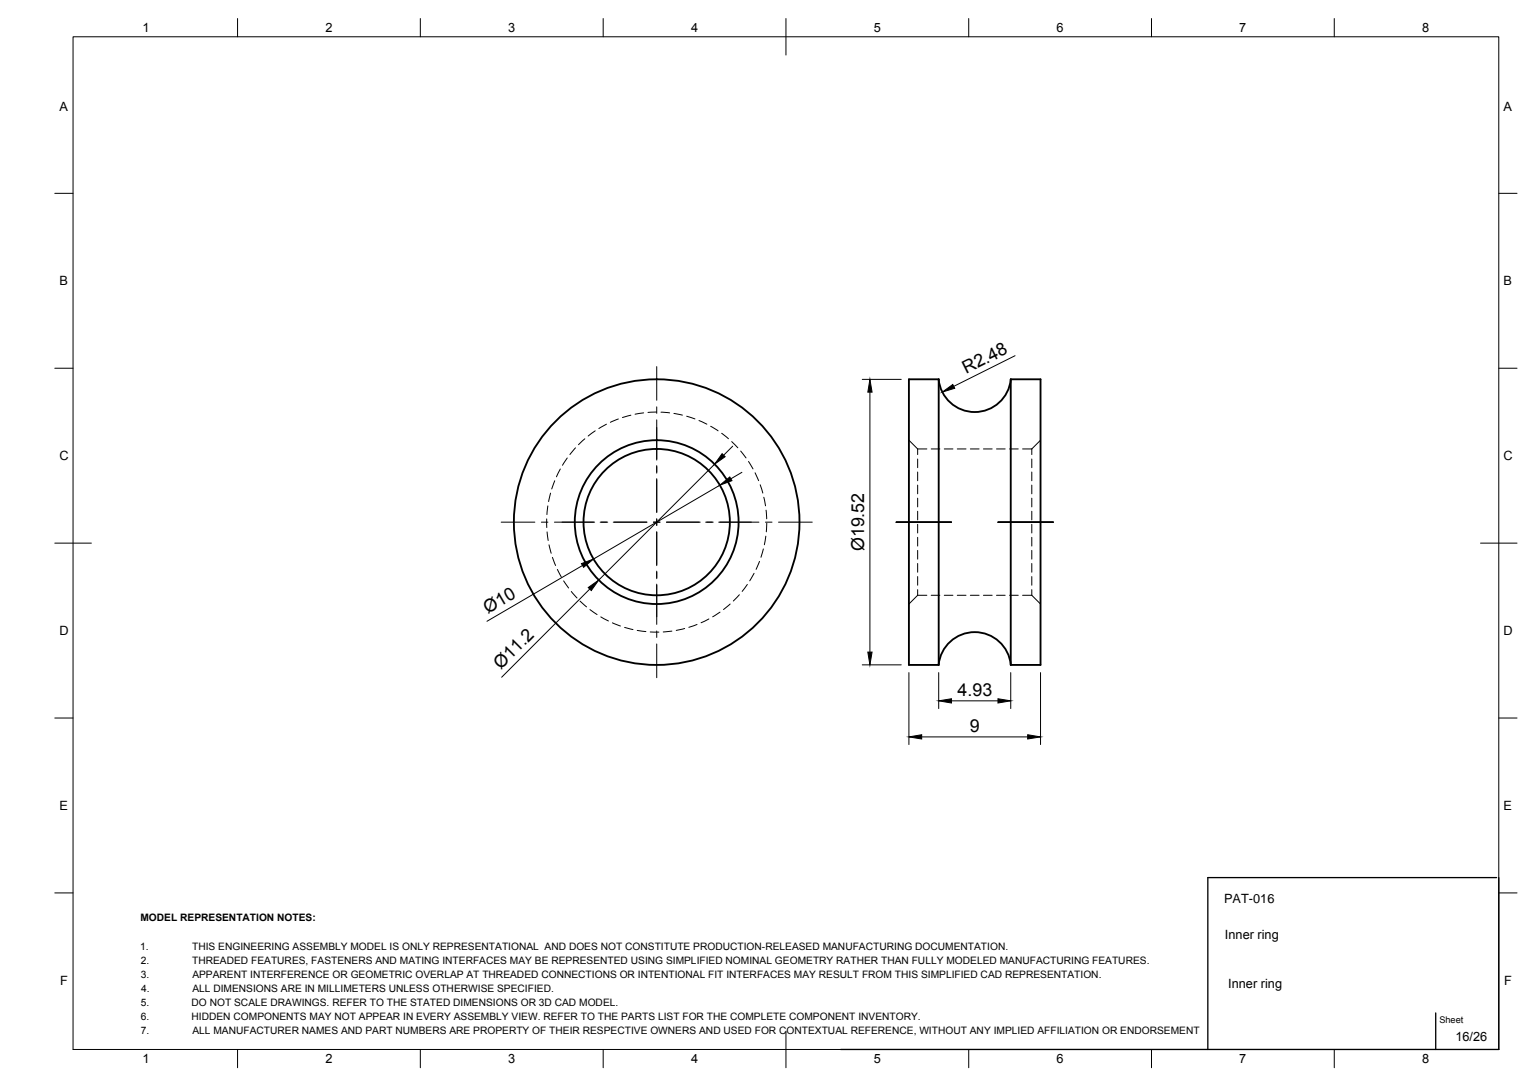
ISO-10303-21;
HEADER;
/* Generated by software containing ST-Developer
 * from STEP Tools, Inc. (www.steptools.com) 
 */

FILE_DESCRIPTION(
/* description */ ('Bracket-mounted idler roller'),
/* implementation_level */ '2;1');

FILE_NAME(
/* name */ 'Inner ring.step',
/* time_stamp */ '2026-10-28T03:26:42-07:00',
/* author */ (''),
/* organization */ (''),
/* preprocessor_version */ 'ST-DEVELOPER v20.2',
/* originating_system */ 'Autodesk Translation Framework v15.17.0.0',
/* authorisation */ '');

FILE_SCHEMA (('AUTOMOTIVE_DESIGN { 1 0 10303 214 3 1 1 }'));
ENDSEC;

DATA;
#10=MECHANICAL_DESIGN_GEOMETRIC_PRESENTATION_REPRESENTATION('',(#291),#6241);
#221=TOROIDAL_SURFACE('',#3608,1.,0.247676);
#226=CONICAL_SURFACE('',#3619,0.53,0.785398163397448);
#227=CONICAL_SURFACE('',#3626,0.53,0.785398163397448);
#249=SHAPE_REPRESENTATION_RELATIONSHIP('SRR','None',#6354,#270);
#270=ADVANCED_BREP_SHAPE_REPRESENTATION('',(#319),#6230);
#291=STYLED_ITEM('',(#6538),#319);
#319=MANIFOLD_SOLID_BREP('Body1',#3194);
#373=FACE_BOUND('',#840,.T.);
#374=FACE_BOUND('',#843,.T.);
#478=PLANE('',#3621);
#479=PLANE('',#3624);
#607=FACE_OUTER_BOUND('',#835,.T.);
#608=FACE_OUTER_BOUND('',#836,.T.);
#609=FACE_OUTER_BOUND('',#837,.T.);
#610=FACE_OUTER_BOUND('',#838,.T.);
#611=FACE_OUTER_BOUND('',#839,.T.);
#612=FACE_OUTER_BOUND('',#841,.T.);
#613=FACE_OUTER_BOUND('',#842,.T.);
#614=FACE_OUTER_BOUND('',#844,.T.);
#835=EDGE_LOOP('',(#2520,#2521,#2522,#2523,#2524,#2525));
#836=EDGE_LOOP('',(#2526,#2527,#2528,#2529,#2530));
#837=EDGE_LOOP('',(#2531,#2532,#2533,#2534));
#838=EDGE_LOOP('',(#2535,#2536,#2537,#2538));
#839=EDGE_LOOP('',(#2539));
#840=EDGE_LOOP('',(#2540));
#841=EDGE_LOOP('',(#2541,#2542,#2543,#2544,#2545));
#842=EDGE_LOOP('',(#2546));
#843=EDGE_LOOP('',(#2547));
#844=EDGE_LOOP('',(#2548,#2549,#2550,#2551));
#1099=LINE('',#5362,#1281);
#1100=LINE('',#5368,#1282);
#1101=LINE('',#5372,#1283);
#1102=LINE('',#5378,#1284);
#1103=LINE('',#5383,#1285);
#1281=VECTOR('',#4346,0.976185);
#1282=VECTOR('',#4353,0.5);
#1283=VECTOR('',#4358,0.53);
#1284=VECTOR('',#4367,0.976185);
#1285=VECTOR('',#4374,0.53);
#1400=CIRCLE('',#3609,0.976185);
#1401=CIRCLE('',#3610,0.976185);
#1402=CIRCLE('',#3611,0.247676);
#1403=CIRCLE('',#3612,0.976185);
#1404=CIRCLE('',#3613,0.976185);
#1405=CIRCLE('',#3615,0.976185);
#1406=CIRCLE('',#3617,0.5);
#1407=CIRCLE('',#3618,0.5);
#1408=CIRCLE('',#3620,0.56);
#1409=CIRCLE('',#3623,0.976185);
#1410=CIRCLE('',#3625,0.56);
#1641=VERTEX_POINT('',#5351);
#1642=VERTEX_POINT('',#5352);
#1643=VERTEX_POINT('',#5355);
#1644=VERTEX_POINT('',#5357);
#1645=VERTEX_POINT('',#5361);
#1646=VERTEX_POINT('',#5365);
#1647=VERTEX_POINT('',#5367);
#1648=VERTEX_POINT('',#5371);
#1649=VERTEX_POINT('',#5376);
#1650=VERTEX_POINT('',#5380);
#1962=EDGE_CURVE('',#1641,#1642,#1400,.T.);
#1963=EDGE_CURVE('',#1642,#1641,#1401,.T.);
#1964=EDGE_CURVE('',#1642,#1643,#1402,.T.);
#1965=EDGE_CURVE('',#1644,#1643,#1403,.T.);
#1966=EDGE_CURVE('',#1643,#1644,#1404,.T.);
#1967=EDGE_CURVE('',#1644,#1645,#1099,.T.);
#1968=EDGE_CURVE('',#1645,#1645,#1405,.T.);
#1969=EDGE_CURVE('',#1646,#1646,#1406,.T.);
#1970=EDGE_CURVE('',#1646,#1647,#1100,.T.);
#1971=EDGE_CURVE('',#1647,#1647,#1407,.T.);
#1972=EDGE_CURVE('',#1647,#1648,#1101,.T.);
#1973=EDGE_CURVE('',#1648,#1648,#1408,.T.);
#1974=EDGE_CURVE('',#1649,#1649,#1409,.T.);
#1975=EDGE_CURVE('',#1649,#1641,#1102,.T.);
#1976=EDGE_CURVE('',#1650,#1650,#1410,.T.);
#1977=EDGE_CURVE('',#1650,#1646,#1103,.T.);
#2520=ORIENTED_EDGE('',*,*,#1962,.F.);
#2521=ORIENTED_EDGE('',*,*,#1963,.F.);
#2522=ORIENTED_EDGE('',*,*,#1964,.T.);
#2523=ORIENTED_EDGE('',*,*,#1965,.F.);
#2524=ORIENTED_EDGE('',*,*,#1966,.F.);
#2525=ORIENTED_EDGE('',*,*,#1964,.F.);
#2526=ORIENTED_EDGE('',*,*,#1965,.T.);
#2527=ORIENTED_EDGE('',*,*,#1966,.T.);
#2528=ORIENTED_EDGE('',*,*,#1967,.T.);
#2529=ORIENTED_EDGE('',*,*,#1968,.T.);
#2530=ORIENTED_EDGE('',*,*,#1967,.F.);
#2531=ORIENTED_EDGE('',*,*,#1969,.T.);
#2532=ORIENTED_EDGE('',*,*,#1970,.T.);
#2533=ORIENTED_EDGE('',*,*,#1971,.F.);
#2534=ORIENTED_EDGE('',*,*,#1970,.F.);
#2535=ORIENTED_EDGE('',*,*,#1971,.T.);
#2536=ORIENTED_EDGE('',*,*,#1972,.T.);
#2537=ORIENTED_EDGE('',*,*,#1973,.F.);
#2538=ORIENTED_EDGE('',*,*,#1972,.F.);
#2539=ORIENTED_EDGE('',*,*,#1968,.F.);
#2540=ORIENTED_EDGE('',*,*,#1973,.T.);
#2541=ORIENTED_EDGE('',*,*,#1974,.F.);
#2542=ORIENTED_EDGE('',*,*,#1975,.T.);
#2543=ORIENTED_EDGE('',*,*,#1962,.T.);
#2544=ORIENTED_EDGE('',*,*,#1963,.T.);
#2545=ORIENTED_EDGE('',*,*,#1975,.F.);
#2546=ORIENTED_EDGE('',*,*,#1974,.T.);
#2547=ORIENTED_EDGE('',*,*,#1976,.F.);
#2548=ORIENTED_EDGE('',*,*,#1976,.T.);
#2549=ORIENTED_EDGE('',*,*,#1977,.T.);
#2550=ORIENTED_EDGE('',*,*,#1969,.F.);
#2551=ORIENTED_EDGE('',*,*,#1977,.F.);
#2955=CYLINDRICAL_SURFACE('',#3614,0.976185);
#2956=CYLINDRICAL_SURFACE('',#3616,0.5);
#2957=CYLINDRICAL_SURFACE('',#3622,0.976185);
#3082=ADVANCED_FACE('',(#607),#221,.F.);
#3083=ADVANCED_FACE('',(#608),#2955,.T.);
#3084=ADVANCED_FACE('',(#609),#2956,.F.);
#3085=ADVANCED_FACE('',(#610),#226,.F.);
#3086=ADVANCED_FACE('',(#611,#373),#478,.T.);
#3087=ADVANCED_FACE('',(#612),#2957,.T.);
#3088=ADVANCED_FACE('',(#613,#374),#479,.T.);
#3089=ADVANCED_FACE('',(#614),#227,.F.);
#3194=CLOSED_SHELL('',(#3082,#3083,#3084,#3085,#3086,#3087,#3088,#3089));
#3607=AXIS2_PLACEMENT_3D('',#5349,#4330,#4331);
#3608=AXIS2_PLACEMENT_3D('',#5350,#4332,#4333);
#3609=AXIS2_PLACEMENT_3D('',#5353,#4334,#4335);
#3610=AXIS2_PLACEMENT_3D('',#5354,#4336,#4337);
#3611=AXIS2_PLACEMENT_3D('',#5356,#4338,#4339);
#3612=AXIS2_PLACEMENT_3D('',#5358,#4340,#4341);
#3613=AXIS2_PLACEMENT_3D('',#5359,#4342,#4343);
#3614=AXIS2_PLACEMENT_3D('',#5360,#4344,#4345);
#3615=AXIS2_PLACEMENT_3D('',#5363,#4347,#4348);
#3616=AXIS2_PLACEMENT_3D('',#5364,#4349,#4350);
#3617=AXIS2_PLACEMENT_3D('',#5366,#4351,#4352);
#3618=AXIS2_PLACEMENT_3D('',#5369,#4354,#4355);
#3619=AXIS2_PLACEMENT_3D('',#5370,#4356,#4357);
#3620=AXIS2_PLACEMENT_3D('',#5373,#4359,#4360);
#3621=AXIS2_PLACEMENT_3D('',#5374,#4361,#4362);
#3622=AXIS2_PLACEMENT_3D('',#5375,#4363,#4364);
#3623=AXIS2_PLACEMENT_3D('',#5377,#4365,#4366);
#3624=AXIS2_PLACEMENT_3D('',#5379,#4368,#4369);
#3625=AXIS2_PLACEMENT_3D('',#5381,#4370,#4371);
#3626=AXIS2_PLACEMENT_3D('',#5382,#4372,#4373);
#4330=DIRECTION('axis',(0.,0.,1.));
#4331=DIRECTION('refdir',(1.,0.,0.));
#4332=DIRECTION('center_axis',(0.,-1.,0.));
#4333=DIRECTION('ref_axis',(0.,0.,-1.));
#4334=DIRECTION('center_axis',(0.,-1.,0.));
#4335=DIRECTION('ref_axis',(1.,0.,0.));
#4336=DIRECTION('center_axis',(0.,-1.,0.));
#4337=DIRECTION('ref_axis',(1.,0.,0.));
#4338=DIRECTION('center_axis',(1.,0.,1.22464679914735E-16));
#4339=DIRECTION('ref_axis',(-1.22464679914735E-16,0.,1.));
#4340=DIRECTION('center_axis',(0.,1.,0.));
#4341=DIRECTION('ref_axis',(1.,0.,0.));
#4342=DIRECTION('center_axis',(0.,1.,0.));
#4343=DIRECTION('ref_axis',(1.,0.,0.));
#4344=DIRECTION('center_axis',(0.,-1.,0.));
#4345=DIRECTION('ref_axis',(1.,0.,0.));
#4346=DIRECTION('',(0.,1.,0.));
#4347=DIRECTION('center_axis',(0.,-1.,0.));
#4348=DIRECTION('ref_axis',(1.,0.,0.));
#4349=DIRECTION('center_axis',(0.,-1.,0.));
#4350=DIRECTION('ref_axis',(1.,0.,0.));
#4351=DIRECTION('center_axis',(0.,-1.,0.));
#4352=DIRECTION('ref_axis',(1.,0.,0.));
#4353=DIRECTION('',(0.,1.,0.));
#4354=DIRECTION('center_axis',(0.,-1.,0.));
#4355=DIRECTION('ref_axis',(1.,0.,0.));
#4356=DIRECTION('center_axis',(0.,1.,0.));
#4357=DIRECTION('ref_axis',(1.,0.,0.));
#4358=DIRECTION('',(-0.707106781186547,0.707106781186548,-8.65956056235493E-17));
#4359=DIRECTION('center_axis',(0.,-1.,0.));
#4360=DIRECTION('ref_axis',(1.,0.,0.));
#4361=DIRECTION('center_axis',(0.,1.,0.));
#4362=DIRECTION('ref_axis',(0.,0.,1.));
#4363=DIRECTION('center_axis',(0.,-1.,0.));
#4364=DIRECTION('ref_axis',(1.,0.,0.));
#4365=DIRECTION('center_axis',(0.,-1.,0.));
#4366=DIRECTION('ref_axis',(1.,0.,0.));
#4367=DIRECTION('',(0.,1.,0.));
#4368=DIRECTION('center_axis',(0.,-1.,0.));
#4369=DIRECTION('ref_axis',(0.,0.,-1.));
#4370=DIRECTION('center_axis',(0.,-1.,0.));
#4371=DIRECTION('ref_axis',(1.,0.,0.));
#4372=DIRECTION('center_axis',(0.,-1.,0.));
#4373=DIRECTION('ref_axis',(1.,0.,0.));
#4374=DIRECTION('',(0.707106781186547,0.707106781186548,8.65956056235493E-17));
#5349=CARTESIAN_POINT('',(0.,0.,0.));
#5350=CARTESIAN_POINT('Origin',(0.,0.,0.));
#5351=CARTESIAN_POINT('',(-0.976185,-0.246528389340863,-1.19548183562566E-16));
#5352=CARTESIAN_POINT('',(-1.19548183562566E-16,-0.246528389340863,0.976185));
#5353=CARTESIAN_POINT('Origin',(0.,-0.246528389340863,0.));
#5354=CARTESIAN_POINT('Origin',(0.,-0.246528389340863,0.));
#5355=CARTESIAN_POINT('',(-1.19548183562566E-16,0.246528389340863,0.976185));
#5356=CARTESIAN_POINT('Origin',(-1.22464679914735E-16,0.,1.));
#5357=CARTESIAN_POINT('',(-0.976185,0.246528389340863,1.19548183562566E-16));
#5358=CARTESIAN_POINT('Origin',(0.,0.246528389340863,0.));
#5359=CARTESIAN_POINT('Origin',(0.,0.246528389340863,0.));
#5360=CARTESIAN_POINT('Origin',(0.,0.,0.));
#5361=CARTESIAN_POINT('',(-0.976185,0.45,-1.19548183562566E-16));
#5362=CARTESIAN_POINT('',(-0.976185,0.,-1.19548183562566E-16));
#5363=CARTESIAN_POINT('Origin',(0.,0.45,0.));
#5364=CARTESIAN_POINT('Origin',(0.,0.,0.));
#5365=CARTESIAN_POINT('',(-0.5,-0.39,-6.12323399573677E-17));
#5366=CARTESIAN_POINT('Origin',(0.,-0.39,0.));
#5367=CARTESIAN_POINT('',(-0.5,0.39,-6.12323399573677E-17));
#5368=CARTESIAN_POINT('',(-0.5,0.,-6.12323399573677E-17));
#5369=CARTESIAN_POINT('Origin',(0.,0.39,0.));
#5370=CARTESIAN_POINT('Origin',(0.,0.42,0.));
#5371=CARTESIAN_POINT('',(-0.56,0.45,-6.85802207522518E-17));
#5372=CARTESIAN_POINT('',(-0.53,0.42,-6.49062803548097E-17));
#5373=CARTESIAN_POINT('Origin',(0.,0.45,0.));
#5374=CARTESIAN_POINT('Origin',(0.976185,0.45,0.));
#5375=CARTESIAN_POINT('Origin',(0.,0.,0.));
#5376=CARTESIAN_POINT('',(-0.976185,-0.45,-1.19548183562566E-16));
#5377=CARTESIAN_POINT('Origin',(0.,-0.45,0.));
#5378=CARTESIAN_POINT('',(-0.976185,0.,-1.19548183562566E-16));
#5379=CARTESIAN_POINT('Origin',(0.56,-0.45,0.));
#5380=CARTESIAN_POINT('',(-0.56,-0.45,-6.85802207522518E-17));
#5381=CARTESIAN_POINT('Origin',(0.,-0.45,0.));
#5382=CARTESIAN_POINT('Origin',(0.,-0.42,0.));
#5383=CARTESIAN_POINT('',(-0.53,-0.42,-6.49062803548097E-17));
#6204=UNCERTAINTY_MEASURE_WITH_UNIT(LENGTH_MEASURE(0.001),#6242,
'DISTANCE_ACCURACY_VALUE',
'Maximum model space distance between geometric entities at asserted c
onnectivities');
#6215=UNCERTAINTY_MEASURE_WITH_UNIT(LENGTH_MEASURE(0.001),#6242,
'DISTANCE_ACCURACY_VALUE',
'Maximum model space distance between geometric entities at asserted c
onnectivities');
#6230=(
GEOMETRIC_REPRESENTATION_CONTEXT(3)
GLOBAL_UNCERTAINTY_ASSIGNED_CONTEXT((#6204))
GLOBAL_UNIT_ASSIGNED_CONTEXT((#6242,#6244,#6245))
REPRESENTATION_CONTEXT('','3D')
);
#6241=(
GEOMETRIC_REPRESENTATION_CONTEXT(3)
GLOBAL_UNCERTAINTY_ASSIGNED_CONTEXT((#6215))
GLOBAL_UNIT_ASSIGNED_CONTEXT((#6242,#6244,#6245))
REPRESENTATION_CONTEXT('','3D')
);
#6242=(
LENGTH_UNIT()
NAMED_UNIT(*)
SI_UNIT(.CENTI.,.METRE.)
);
#6244=(
NAMED_UNIT(*)
PLANE_ANGLE_UNIT()
SI_UNIT($,.RADIAN.)
);
#6245=(
NAMED_UNIT(*)
SI_UNIT($,.STERADIAN.)
SOLID_ANGLE_UNIT()
);
#6260=SHAPE_DEFINITION_REPRESENTATION(#6285,#6354);
#6285=PRODUCT_DEFINITION_SHAPE('',$,#6380);
#6354=SHAPE_REPRESENTATION('',(#3607),#6230);
#6365=PRODUCT_DEFINITION_CONTEXT('part definition',#6442,'design');
#6380=PRODUCT_DEFINITION('Inner ring','Inner ring',#6405,#6365);
#6405=PRODUCT_DEFINITION_FORMATION('',$,#6458);
#6442=APPLICATION_CONTEXT(
'Core Data for Automotive Mechanical Design Process');
#6443=PRODUCT_CONTEXT('part definition',#6442,'mechanical');
#6458=PRODUCT('Inner ring','Inner ring','Inner ring',(#6443));
#6532=COLOUR_RGB('Grey',0.48,0.52,0.57);
#6533=FILL_AREA_STYLE_COLOUR('',#6532);
#6534=FILL_AREA_STYLE('',(#6533));
#6535=SURFACE_STYLE_FILL_AREA(#6534);
#6536=SURFACE_SIDE_STYLE('',(#6535));
#6537=SURFACE_STYLE_USAGE(.BOTH.,#6536);
#6538=PRESENTATION_STYLE_ASSIGNMENT((#6537));
ENDSEC;
END-ISO-10303-21;
